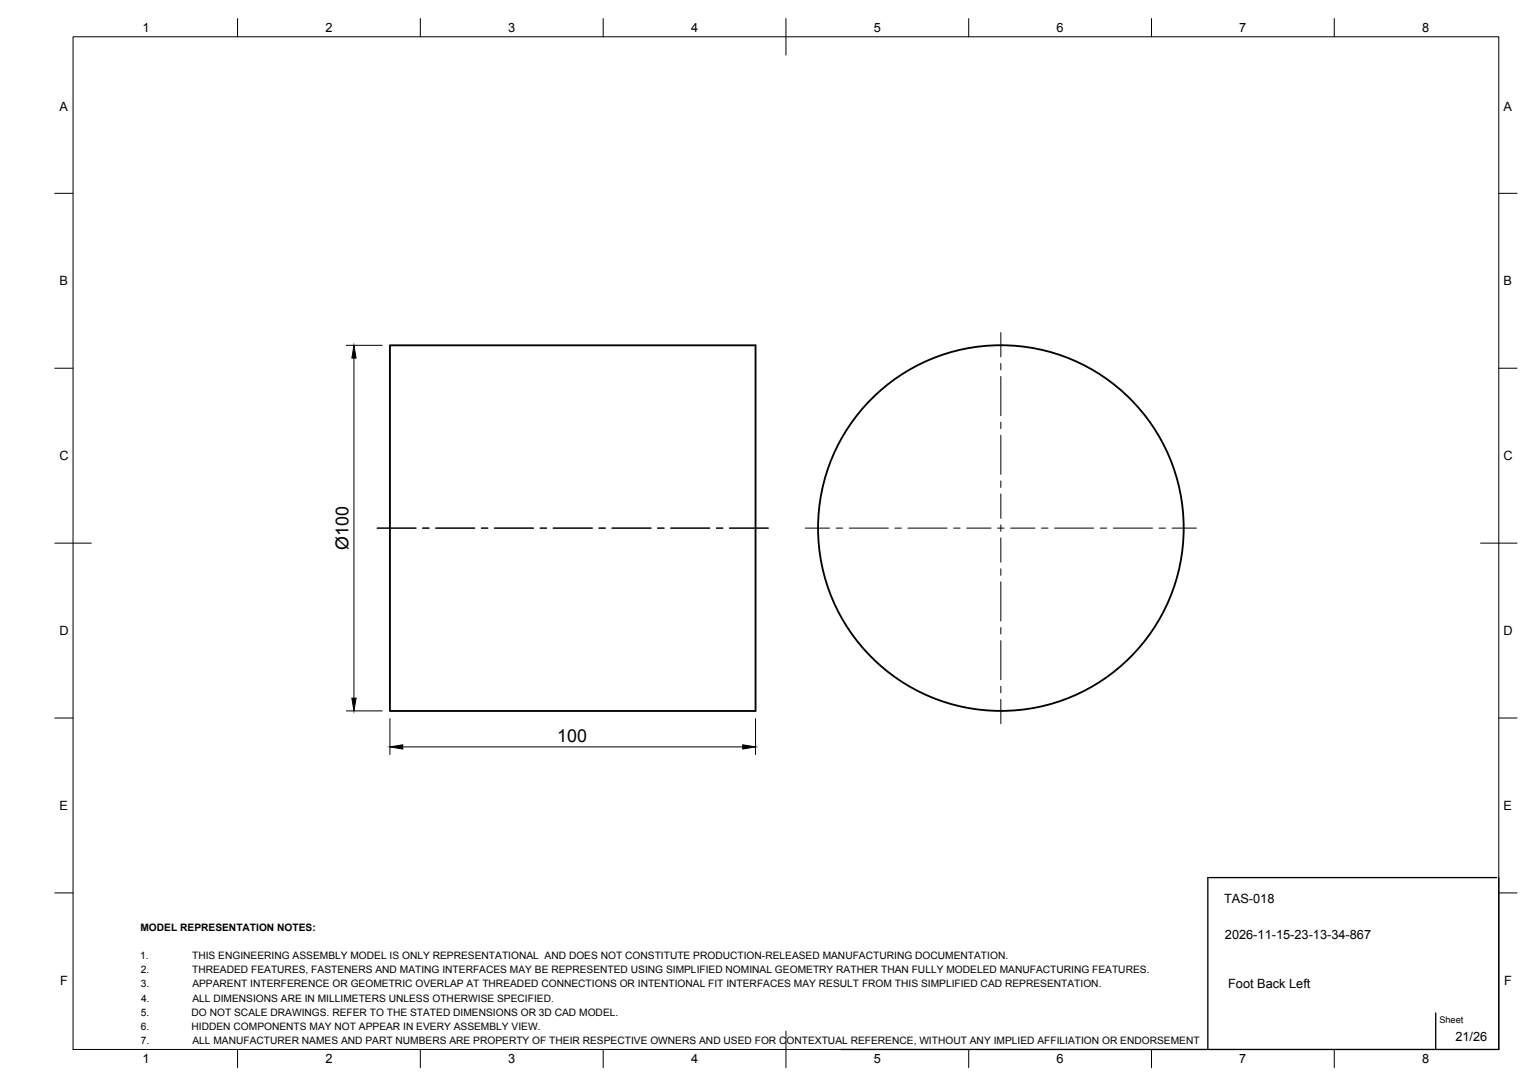
ISO-10303-21;
HEADER;
/* Generated by software containing ST-Developer
 * from STEP Tools, Inc. (www.steptools.com) 
 */

FILE_DESCRIPTION(
/* description */ (''),
/* implementation_level */ '2;1');

FILE_NAME(
/* name */ 'Foot Back Left.step',
/* time_stamp */ '2026-11-15T15:17:57-08:00',
/* author */ (''),
/* organization */ (''),
/* preprocessor_version */ 'ST-DEVELOPER v20.2',
/* originating_system */ 'Autodesk Translation Framework v15.17.0.0',
/* authorisation */ '');

FILE_SCHEMA (('AUTOMOTIVE_DESIGN { 1 0 10303 214 3 1 1 }'));
ENDSEC;

DATA;
#10=MECHANICAL_DESIGN_GEOMETRIC_PRESENTATION_REPRESENTATION('',(#196),#3723);
#19=CIRCLE('',#2448,1.96850393700787);
#20=CIRCLE('',#2449,1.96850393700787);
#27=CYLINDRICAL_SURFACE('',#2447,1.96850393700787);
#148=SHAPE_REPRESENTATION_RELATIONSHIP('SRR','None',#3829,#172);
#172=ADVANCED_BREP_SHAPE_REPRESENTATION('',(#220),#3718);
#196=STYLED_ITEM('',(#3945),#220);
#220=MANIFOLD_SOLID_BREP('Body1',#2044);
#327=FACE_OUTER_BOUND('',#453,.T.);
#328=FACE_OUTER_BOUND('',#454,.T.);
#329=FACE_OUTER_BOUND('',#455,.T.);
#453=EDGE_LOOP('',(#1695,#1696,#1697,#1698));
#454=EDGE_LOOP('',(#1699));
#455=EDGE_LOOP('',(#1700));
#661=LINE('',#3552,#883);
#883=VECTOR('',#2957,1.96850393700787);
#1049=VERTEX_POINT('',#3549);
#1050=VERTEX_POINT('',#3551);
#1269=EDGE_CURVE('',#1049,#1049,#19,.T.);
#1270=EDGE_CURVE('',#1049,#1050,#661,.T.);
#1271=EDGE_CURVE('',#1050,#1050,#20,.T.);
#1695=ORIENTED_EDGE('',*,*,#1269,.T.);
#1696=ORIENTED_EDGE('',*,*,#1270,.T.);
#1697=ORIENTED_EDGE('',*,*,#1271,.F.);
#1698=ORIENTED_EDGE('',*,*,#1270,.F.);
#1699=ORIENTED_EDGE('',*,*,#1271,.T.);
#1700=ORIENTED_EDGE('',*,*,#1269,.F.);
#1877=PLANE('',#2450);
#1878=PLANE('',#2451);
#2001=ADVANCED_FACE('',(#327),#27,.T.);
#2002=ADVANCED_FACE('',(#328),#1877,.T.);
#2003=ADVANCED_FACE('',(#329),#1878,.F.);
#2044=CLOSED_SHELL('',(#2001,#2002,#2003));
#2446=AXIS2_PLACEMENT_3D('',#3547,#2951,#2952);
#2447=AXIS2_PLACEMENT_3D('',#3548,#2953,#2954);
#2448=AXIS2_PLACEMENT_3D('',#3550,#2955,#2956);
#2449=AXIS2_PLACEMENT_3D('',#3553,#2958,#2959);
#2450=AXIS2_PLACEMENT_3D('',#3554,#2960,#2961);
#2451=AXIS2_PLACEMENT_3D('',#3555,#2962,#2963);
#2951=DIRECTION('axis',(0.,0.,1.));
#2952=DIRECTION('refdir',(1.,0.,0.));
#2953=DIRECTION('center_axis',(0.,1.,0.));
#2954=DIRECTION('ref_axis',(0.,0.,1.));
#2955=DIRECTION('center_axis',(0.,-1.,0.));
#2956=DIRECTION('ref_axis',(0.,0.,-1.));
#2957=DIRECTION('',(0.,-1.,0.));
#2958=DIRECTION('center_axis',(0.,-1.,0.));
#2959=DIRECTION('ref_axis',(0.,0.,-1.));
#2960=DIRECTION('center_axis',(0.,-1.,0.));
#2961=DIRECTION('ref_axis',(0.,0.,-1.));
#2962=DIRECTION('center_axis',(0.,-1.,0.));
#2963=DIRECTION('ref_axis',(0.,0.,-1.));
#3547=CARTESIAN_POINT('',(0.,0.,0.));
#3548=CARTESIAN_POINT('Origin',(-33.6377952755905,-4.91732638859567E-15,
2.36220472440945));
#3549=CARTESIAN_POINT('',(-33.6377952755905,3.93700787401574,0.393700787401579));
#3550=CARTESIAN_POINT('Origin',(-33.6377952755905,3.93700787401574,2.36220472440945));
#3551=CARTESIAN_POINT('',(-33.6377952755905,-4.91732638859567E-15,0.393700787401579));
#3552=CARTESIAN_POINT('',(-33.6377952755905,-4.91732638859567E-15,0.393700787401579));
#3553=CARTESIAN_POINT('Origin',(-33.6377952755905,-4.91732638859567E-15,
2.36220472440945));
#3554=CARTESIAN_POINT('Origin',(-33.6377952755905,-4.91732638859567E-15,
2.36220472440945));
#3555=CARTESIAN_POINT('Origin',(-33.6377952755905,3.93700787401574,2.36220472440945));
#3691=UNCERTAINTY_MEASURE_WITH_UNIT(LENGTH_MEASURE(0.000393700787401575),
#3725,'DISTANCE_ACCURACY_VALUE',
'Maximum model space distance between geometric entities at asserted c
onnectivities');
#3696=UNCERTAINTY_MEASURE_WITH_UNIT(LENGTH_MEASURE(0.000393700787401575),
#3725,'DISTANCE_ACCURACY_VALUE',
'Maximum model space distance between geometric entities at asserted c
onnectivities');
#3718=(
GEOMETRIC_REPRESENTATION_CONTEXT(3)
GLOBAL_UNCERTAINTY_ASSIGNED_CONTEXT((#3691))
GLOBAL_UNIT_ASSIGNED_CONTEXT((#3725,#3729,#3730))
REPRESENTATION_CONTEXT('','3D')
);
#3723=(
GEOMETRIC_REPRESENTATION_CONTEXT(3)
GLOBAL_UNCERTAINTY_ASSIGNED_CONTEXT((#3696))
GLOBAL_UNIT_ASSIGNED_CONTEXT((#3725,#3729,#3730))
REPRESENTATION_CONTEXT('','3D')
);
#3724=DIMENSIONAL_EXPONENTS(1.,0.,0.,0.,0.,0.,0.);
#3725=(
CONVERSION_BASED_UNIT('inch',#3728)
LENGTH_UNIT()
NAMED_UNIT(#3724)
);
#3726=(
LENGTH_UNIT()
NAMED_UNIT(*)
SI_UNIT(.MILLI.,.METRE.)
);
#3728=LENGTH_MEASURE_WITH_UNIT(LENGTH_MEASURE(25.4),#3726);
#3729=(
NAMED_UNIT(*)
PLANE_ANGLE_UNIT()
SI_UNIT($,.RADIAN.)
);
#3730=(
NAMED_UNIT(*)
SI_UNIT($,.STERADIAN.)
SOLID_ANGLE_UNIT()
);
#3752=SHAPE_DEFINITION_REPRESENTATION(#3779,#3829);
#3779=PRODUCT_DEFINITION_SHAPE('',$,#3856);
#3829=SHAPE_REPRESENTATION('',(#2446),#3718);
#3834=PRODUCT_DEFINITION_CONTEXT('part definition',#3914,'design');
#3856=PRODUCT_DEFINITION('2026-11-15-23-13-34-867','Foot Back Left',#3882,
#3834);
#3882=PRODUCT_DEFINITION_FORMATION('',$,#3937);
#3914=APPLICATION_CONTEXT(
'Core Data for Automotive Mechanical Design Process');
#3915=PRODUCT_CONTEXT('part definition',#3914,'mechanical');
#3937=PRODUCT('2026-11-15-23-13-34-867','Foot Back Left',$,(#3915));
#3945=PRESENTATION_STYLE_ASSIGNMENT((#3953));
#3953=SURFACE_STYLE_USAGE(.BOTH.,#3961);
#3961=SURFACE_SIDE_STYLE('',(#3969));
#3969=SURFACE_STYLE_FILL_AREA(#3977);
#3977=FILL_AREA_STYLE('Black',(#3985));
#3985=FILL_AREA_STYLE_COLOUR('Black',#3993);
#3993=COLOUR_RGB('Black',0.0784313725490196,0.0784313725490196,0.0784313725490196);
ENDSEC;
END-ISO-10303-21;
